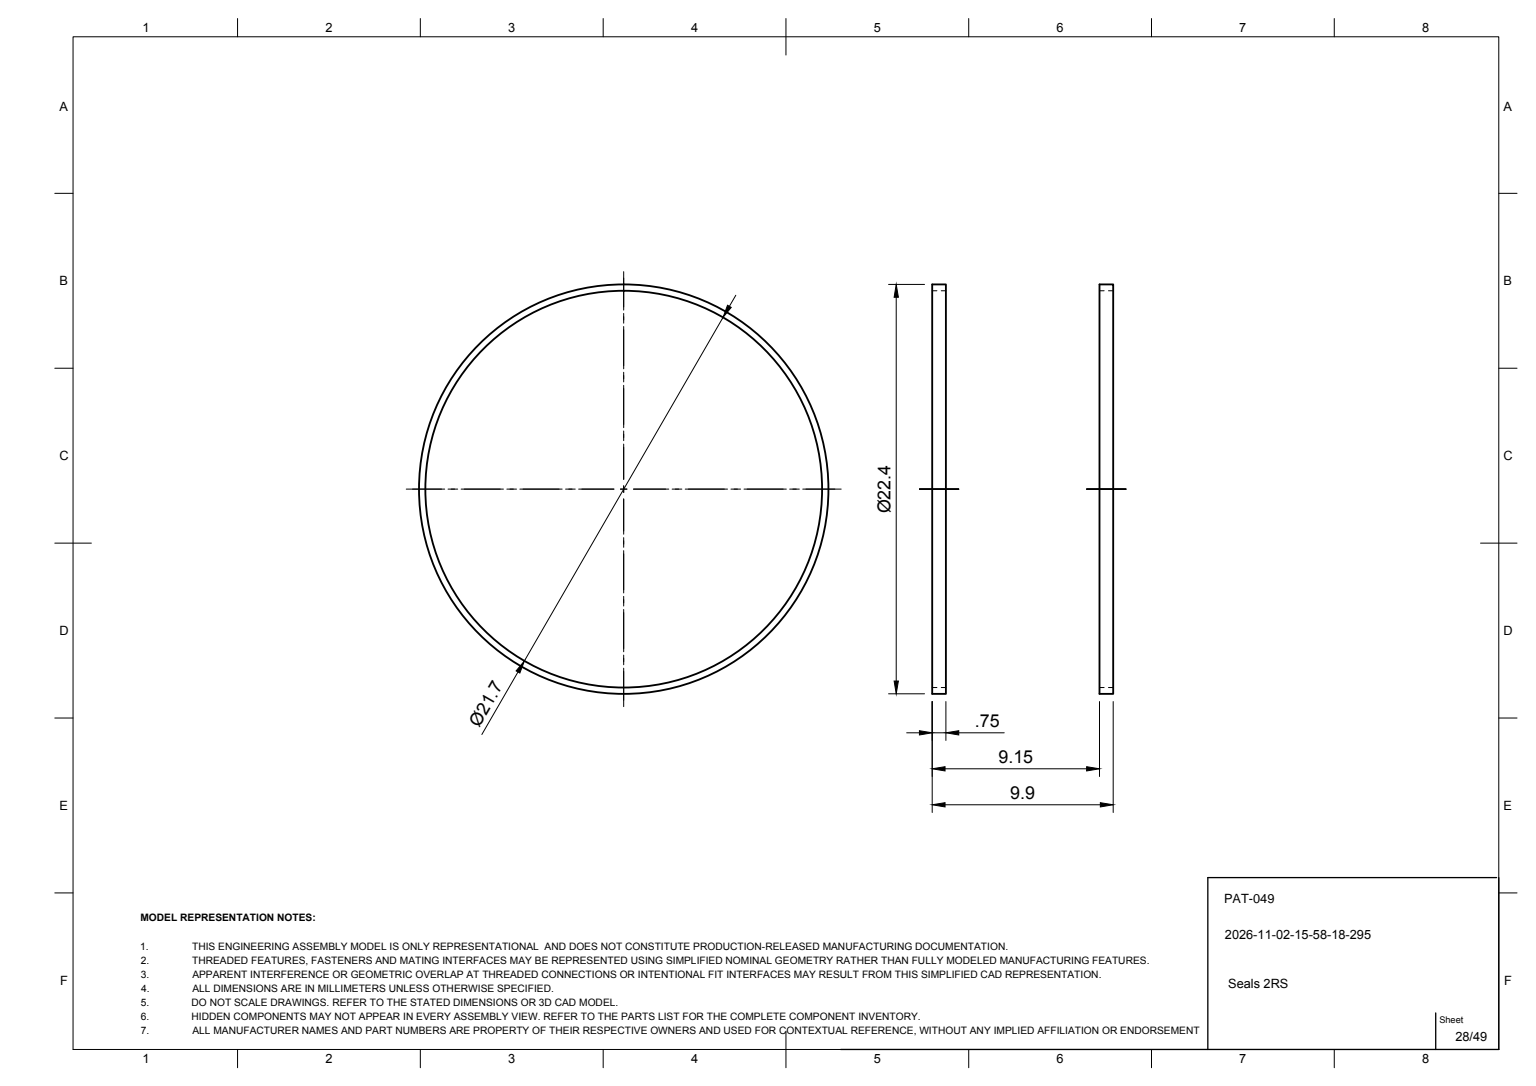
ISO-10303-21;
HEADER;
/* Generated by software containing ST-Developer
 * from STEP Tools, Inc. (www.steptools.com) 
 */

FILE_DESCRIPTION(
/* description */ ('Hand drill press frame (manual)'),
/* implementation_level */ '2;1');

FILE_NAME(
/* name */ 'Seals 2RS.step',
/* time_stamp */ '2026-10-28T03:25:28-07:00',
/* author */ (''),
/* organization */ (''),
/* preprocessor_version */ 'ST-DEVELOPER v20.2',
/* originating_system */ 'Autodesk Translation Framework v15.17.0.0',
/* authorisation */ '');

FILE_SCHEMA (('AUTOMOTIVE_DESIGN { 1 0 10303 214 3 1 1 }'));
ENDSEC;

DATA;
#10=MECHANICAL_DESIGN_GEOMETRIC_PRESENTATION_REPRESENTATION('',(#646,#647),#33299);
#550=SHAPE_REPRESENTATION_RELATIONSHIP('SRR','None',#33510,#595);
#595=ADVANCED_BREP_SHAPE_REPRESENTATION('',(#698,#699),#33272);
#646=STYLED_ITEM('',(#33814),#698);
#647=STYLED_ITEM('',(#33814),#699);
#698=MANIFOLD_SOLID_BREP('Body1',#12664);
#699=MANIFOLD_SOLID_BREP('Body2',#12665);
#841=FACE_BOUND('',#2407,.T.);
#842=FACE_BOUND('',#2410,.T.);
#843=FACE_BOUND('',#2413,.T.);
#844=FACE_BOUND('',#2416,.T.);
#1029=PLANE('',#13710);
#1030=PLANE('',#13715);
#1031=PLANE('',#13718);
#1032=PLANE('',#13723);
#1596=FACE_OUTER_BOUND('',#2406,.T.);
#1597=FACE_OUTER_BOUND('',#2408,.T.);
#1598=FACE_OUTER_BOUND('',#2409,.T.);
#1599=FACE_OUTER_BOUND('',#2411,.T.);
#1600=FACE_OUTER_BOUND('',#2412,.T.);
#1601=FACE_OUTER_BOUND('',#2414,.T.);
#1602=FACE_OUTER_BOUND('',#2415,.T.);
#1603=FACE_OUTER_BOUND('',#2417,.T.);
#2406=EDGE_LOOP('',(#9621));
#2407=EDGE_LOOP('',(#9622));
#2408=EDGE_LOOP('',(#9623,#9624,#9625,#9626));
#2409=EDGE_LOOP('',(#9627));
#2410=EDGE_LOOP('',(#9628));
#2411=EDGE_LOOP('',(#9629,#9630,#9631,#9632));
#2412=EDGE_LOOP('',(#9633));
#2413=EDGE_LOOP('',(#9634));
#2414=EDGE_LOOP('',(#9635,#9636,#9637,#9638));
#2415=EDGE_LOOP('',(#9639));
#2416=EDGE_LOOP('',(#9640));
#2417=EDGE_LOOP('',(#9641,#9642,#9643,#9644));
#3215=LINE('',#19665,#4380);
#3216=LINE('',#19670,#4381);
#3217=LINE('',#19679,#4382);
#3218=LINE('',#19684,#4383);
#4380=VECTOR('',#15752,1.119765);
#4381=VECTOR('',#15759,1.085235);
#4382=VECTOR('',#15770,1.119765);
#4383=VECTOR('',#15777,1.085235);
#5454=CIRCLE('',#13711,1.119765);
#5455=CIRCLE('',#13712,1.085235);
#5456=CIRCLE('',#13714,1.119765);
#5457=CIRCLE('',#13716,1.085235);
#5458=CIRCLE('',#13719,1.119765);
#5459=CIRCLE('',#13720,1.085235);
#5460=CIRCLE('',#13722,1.119765);
#5461=CIRCLE('',#13724,1.085235);
#6021=VERTEX_POINT('',#19658);
#6022=VERTEX_POINT('',#19660);
#6023=VERTEX_POINT('',#19663);
#6024=VERTEX_POINT('',#19667);
#6025=VERTEX_POINT('',#19672);
#6026=VERTEX_POINT('',#19674);
#6027=VERTEX_POINT('',#19677);
#6028=VERTEX_POINT('',#19681);
#7339=EDGE_CURVE('',#6021,#6021,#5454,.T.);
#7340=EDGE_CURVE('',#6022,#6022,#5455,.T.);
#7341=EDGE_CURVE('',#6023,#6023,#5456,.T.);
#7342=EDGE_CURVE('',#6023,#6021,#3215,.T.);
#7343=EDGE_CURVE('',#6024,#6024,#5457,.T.);
#7344=EDGE_CURVE('',#6024,#6022,#3216,.T.);
#7345=EDGE_CURVE('',#6025,#6025,#5458,.T.);
#7346=EDGE_CURVE('',#6026,#6026,#5459,.T.);
#7347=EDGE_CURVE('',#6027,#6027,#5460,.T.);
#7348=EDGE_CURVE('',#6027,#6025,#3217,.T.);
#7349=EDGE_CURVE('',#6028,#6028,#5461,.T.);
#7350=EDGE_CURVE('',#6028,#6026,#3218,.T.);
#9621=ORIENTED_EDGE('',*,*,#7339,.F.);
#9622=ORIENTED_EDGE('',*,*,#7340,.T.);
#9623=ORIENTED_EDGE('',*,*,#7341,.F.);
#9624=ORIENTED_EDGE('',*,*,#7342,.T.);
#9625=ORIENTED_EDGE('',*,*,#7339,.T.);
#9626=ORIENTED_EDGE('',*,*,#7342,.F.);
#9627=ORIENTED_EDGE('',*,*,#7341,.T.);
#9628=ORIENTED_EDGE('',*,*,#7343,.F.);
#9629=ORIENTED_EDGE('',*,*,#7343,.T.);
#9630=ORIENTED_EDGE('',*,*,#7344,.T.);
#9631=ORIENTED_EDGE('',*,*,#7340,.F.);
#9632=ORIENTED_EDGE('',*,*,#7344,.F.);
#9633=ORIENTED_EDGE('',*,*,#7345,.F.);
#9634=ORIENTED_EDGE('',*,*,#7346,.T.);
#9635=ORIENTED_EDGE('',*,*,#7347,.F.);
#9636=ORIENTED_EDGE('',*,*,#7348,.T.);
#9637=ORIENTED_EDGE('',*,*,#7345,.T.);
#9638=ORIENTED_EDGE('',*,*,#7348,.F.);
#9639=ORIENTED_EDGE('',*,*,#7347,.T.);
#9640=ORIENTED_EDGE('',*,*,#7349,.F.);
#9641=ORIENTED_EDGE('',*,*,#7349,.T.);
#9642=ORIENTED_EDGE('',*,*,#7350,.T.);
#9643=ORIENTED_EDGE('',*,*,#7346,.F.);
#9644=ORIENTED_EDGE('',*,*,#7350,.F.);
#11879=CYLINDRICAL_SURFACE('',#13713,1.119765);
#11880=CYLINDRICAL_SURFACE('',#13717,1.085235);
#11881=CYLINDRICAL_SURFACE('',#13721,1.119765);
#11882=CYLINDRICAL_SURFACE('',#13725,1.085235);
#12205=ADVANCED_FACE('',(#1596,#841),#1029,.T.);
#12206=ADVANCED_FACE('',(#1597),#11879,.T.);
#12207=ADVANCED_FACE('',(#1598,#842),#1030,.T.);
#12208=ADVANCED_FACE('',(#1599),#11880,.F.);
#12209=ADVANCED_FACE('',(#1600,#843),#1031,.T.);
#12210=ADVANCED_FACE('',(#1601),#11881,.T.);
#12211=ADVANCED_FACE('',(#1602,#844),#1032,.T.);
#12212=ADVANCED_FACE('',(#1603),#11882,.F.);
#12664=CLOSED_SHELL('',(#12205,#12206,#12207,#12208));
#12665=CLOSED_SHELL('',(#12209,#12210,#12211,#12212));
#13709=AXIS2_PLACEMENT_3D('',#19656,#15740,#15741);
#13710=AXIS2_PLACEMENT_3D('',#19657,#15742,#15743);
#13711=AXIS2_PLACEMENT_3D('',#19659,#15744,#15745);
#13712=AXIS2_PLACEMENT_3D('',#19661,#15746,#15747);
#13713=AXIS2_PLACEMENT_3D('',#19662,#15748,#15749);
#13714=AXIS2_PLACEMENT_3D('',#19664,#15750,#15751);
#13715=AXIS2_PLACEMENT_3D('',#19666,#15753,#15754);
#13716=AXIS2_PLACEMENT_3D('',#19668,#15755,#15756);
#13717=AXIS2_PLACEMENT_3D('',#19669,#15757,#15758);
#13718=AXIS2_PLACEMENT_3D('',#19671,#15760,#15761);
#13719=AXIS2_PLACEMENT_3D('',#19673,#15762,#15763);
#13720=AXIS2_PLACEMENT_3D('',#19675,#15764,#15765);
#13721=AXIS2_PLACEMENT_3D('',#19676,#15766,#15767);
#13722=AXIS2_PLACEMENT_3D('',#19678,#15768,#15769);
#13723=AXIS2_PLACEMENT_3D('',#19680,#15771,#15772);
#13724=AXIS2_PLACEMENT_3D('',#19682,#15773,#15774);
#13725=AXIS2_PLACEMENT_3D('',#19683,#15775,#15776);
#15740=DIRECTION('axis',(0.,0.,1.));
#15741=DIRECTION('refdir',(1.,0.,0.));
#15742=DIRECTION('center_axis',(0.,1.,0.));
#15743=DIRECTION('ref_axis',(0.,0.,1.));
#15744=DIRECTION('center_axis',(0.,-1.,0.));
#15745=DIRECTION('ref_axis',(1.,0.,0.));
#15746=DIRECTION('center_axis',(0.,-1.,0.));
#15747=DIRECTION('ref_axis',(1.,0.,0.));
#15748=DIRECTION('center_axis',(0.,-1.,0.));
#15749=DIRECTION('ref_axis',(1.,0.,0.));
#15750=DIRECTION('center_axis',(0.,-1.,0.));
#15751=DIRECTION('ref_axis',(1.,0.,0.));
#15752=DIRECTION('',(0.,1.,0.));
#15753=DIRECTION('center_axis',(0.,-1.,0.));
#15754=DIRECTION('ref_axis',(0.,0.,-1.));
#15755=DIRECTION('center_axis',(0.,-1.,0.));
#15756=DIRECTION('ref_axis',(1.,0.,0.));
#15757=DIRECTION('center_axis',(0.,-1.,0.));
#15758=DIRECTION('ref_axis',(1.,0.,0.));
#15759=DIRECTION('',(0.,1.,0.));
#15760=DIRECTION('center_axis',(0.,1.,0.));
#15761=DIRECTION('ref_axis',(0.,0.,1.));
#15762=DIRECTION('center_axis',(0.,-1.,0.));
#15763=DIRECTION('ref_axis',(1.,0.,0.));
#15764=DIRECTION('center_axis',(0.,-1.,0.));
#15765=DIRECTION('ref_axis',(1.,0.,0.));
#15766=DIRECTION('center_axis',(0.,-1.,0.));
#15767=DIRECTION('ref_axis',(1.,0.,0.));
#15768=DIRECTION('center_axis',(0.,-1.,0.));
#15769=DIRECTION('ref_axis',(1.,0.,0.));
#15770=DIRECTION('',(0.,1.,0.));
#15771=DIRECTION('center_axis',(0.,-1.,0.));
#15772=DIRECTION('ref_axis',(0.,0.,-1.));
#15773=DIRECTION('center_axis',(0.,-1.,0.));
#15774=DIRECTION('ref_axis',(1.,0.,0.));
#15775=DIRECTION('center_axis',(0.,-1.,0.));
#15776=DIRECTION('ref_axis',(1.,0.,0.));
#15777=DIRECTION('',(0.,1.,0.));
#19656=CARTESIAN_POINT('',(0.,0.,0.));
#19657=CARTESIAN_POINT('Origin',(1.119765,0.495,0.));
#19658=CARTESIAN_POINT('',(-1.119765,0.495,-1.37131662304724E-16));
#19659=CARTESIAN_POINT('Origin',(0.,0.495,0.));
#19660=CARTESIAN_POINT('',(-1.085235,0.495,-1.32902956907268E-16));
#19661=CARTESIAN_POINT('Origin',(0.,0.495,0.));
#19662=CARTESIAN_POINT('Origin',(0.,0.4575,0.));
#19663=CARTESIAN_POINT('',(-1.119765,0.42,-1.37131662304724E-16));
#19664=CARTESIAN_POINT('Origin',(0.,0.42,0.));
#19665=CARTESIAN_POINT('',(-1.119765,0.4575,-1.37131662304724E-16));
#19666=CARTESIAN_POINT('Origin',(1.085235,0.42,0.));
#19667=CARTESIAN_POINT('',(-1.085235,0.42,-1.32902956907268E-16));
#19668=CARTESIAN_POINT('Origin',(0.,0.42,0.));
#19669=CARTESIAN_POINT('Origin',(0.,0.4575,0.));
#19670=CARTESIAN_POINT('',(-1.085235,0.4575,-1.32902956907268E-16));
#19671=CARTESIAN_POINT('Origin',(1.119765,-0.42,0.));
#19672=CARTESIAN_POINT('',(-1.119765,-0.42,-1.37131662304724E-16));
#19673=CARTESIAN_POINT('Origin',(0.,-0.42,0.));
#19674=CARTESIAN_POINT('',(-1.085235,-0.42,-1.32902956907268E-16));
#19675=CARTESIAN_POINT('Origin',(0.,-0.42,0.));
#19676=CARTESIAN_POINT('Origin',(0.,-0.4575,0.));
#19677=CARTESIAN_POINT('',(-1.119765,-0.495,-1.37131662304724E-16));
#19678=CARTESIAN_POINT('Origin',(0.,-0.495,0.));
#19679=CARTESIAN_POINT('',(-1.119765,-0.4575,-1.37131662304724E-16));
#19680=CARTESIAN_POINT('Origin',(1.085235,-0.495,0.));
#19681=CARTESIAN_POINT('',(-1.085235,-0.495,-1.32902956907268E-16));
#19682=CARTESIAN_POINT('Origin',(0.,-0.495,0.));
#19683=CARTESIAN_POINT('Origin',(0.,-0.4575,0.));
#19684=CARTESIAN_POINT('',(-1.085235,-0.4575,-1.32902956907268E-16));
#33220=UNCERTAINTY_MEASURE_WITH_UNIT(LENGTH_MEASURE(0.001),#33300,
'DISTANCE_ACCURACY_VALUE',
'Maximum model space distance between geometric entities at asserted c
onnectivities');
#33247=UNCERTAINTY_MEASURE_WITH_UNIT(LENGTH_MEASURE(0.001),#33300,
'DISTANCE_ACCURACY_VALUE',
'Maximum model space distance between geometric entities at asserted c
onnectivities');
#33272=(
GEOMETRIC_REPRESENTATION_CONTEXT(3)
GLOBAL_UNCERTAINTY_ASSIGNED_CONTEXT((#33220))
GLOBAL_UNIT_ASSIGNED_CONTEXT((#33300,#33302,#33303))
REPRESENTATION_CONTEXT('','3D')
);
#33299=(
GEOMETRIC_REPRESENTATION_CONTEXT(3)
GLOBAL_UNCERTAINTY_ASSIGNED_CONTEXT((#33247))
GLOBAL_UNIT_ASSIGNED_CONTEXT((#33300,#33302,#33303))
REPRESENTATION_CONTEXT('','3D')
);
#33300=(
LENGTH_UNIT()
NAMED_UNIT(*)
SI_UNIT(.CENTI.,.METRE.)
);
#33302=(
NAMED_UNIT(*)
PLANE_ANGLE_UNIT()
SI_UNIT($,.RADIAN.)
);
#33303=(
NAMED_UNIT(*)
SI_UNIT($,.STERADIAN.)
SOLID_ANGLE_UNIT()
);
#33328=SHAPE_DEFINITION_REPRESENTATION(#33379,#33510);
#33379=PRODUCT_DEFINITION_SHAPE('',$,#33562);
#33510=SHAPE_REPRESENTATION('',(#13709),#33272);
#33537=PRODUCT_DEFINITION_CONTEXT('part definition',#33692,'design');
#33562=PRODUCT_DEFINITION('Seals 2RS','Seals 2RS',#33613,#33537);
#33613=PRODUCT_DEFINITION_FORMATION('',$,#33718);
#33692=APPLICATION_CONTEXT(
'Core Data for Automotive Mechanical Design Process');
#33693=PRODUCT_CONTEXT('part definition',#33692,'mechanical');
#33718=PRODUCT('Seals 2RS','Seals 2RS','Seals 2RS',(#33693));
#33808=COLOUR_RGB('Grey',0.48,0.52,0.57);
#33809=FILL_AREA_STYLE_COLOUR('',#33808);
#33810=FILL_AREA_STYLE('',(#33809));
#33811=SURFACE_STYLE_FILL_AREA(#33810);
#33812=SURFACE_SIDE_STYLE('',(#33811));
#33813=SURFACE_STYLE_USAGE(.BOTH.,#33812);
#33814=PRESENTATION_STYLE_ASSIGNMENT((#33813));
ENDSEC;
END-ISO-10303-21;
